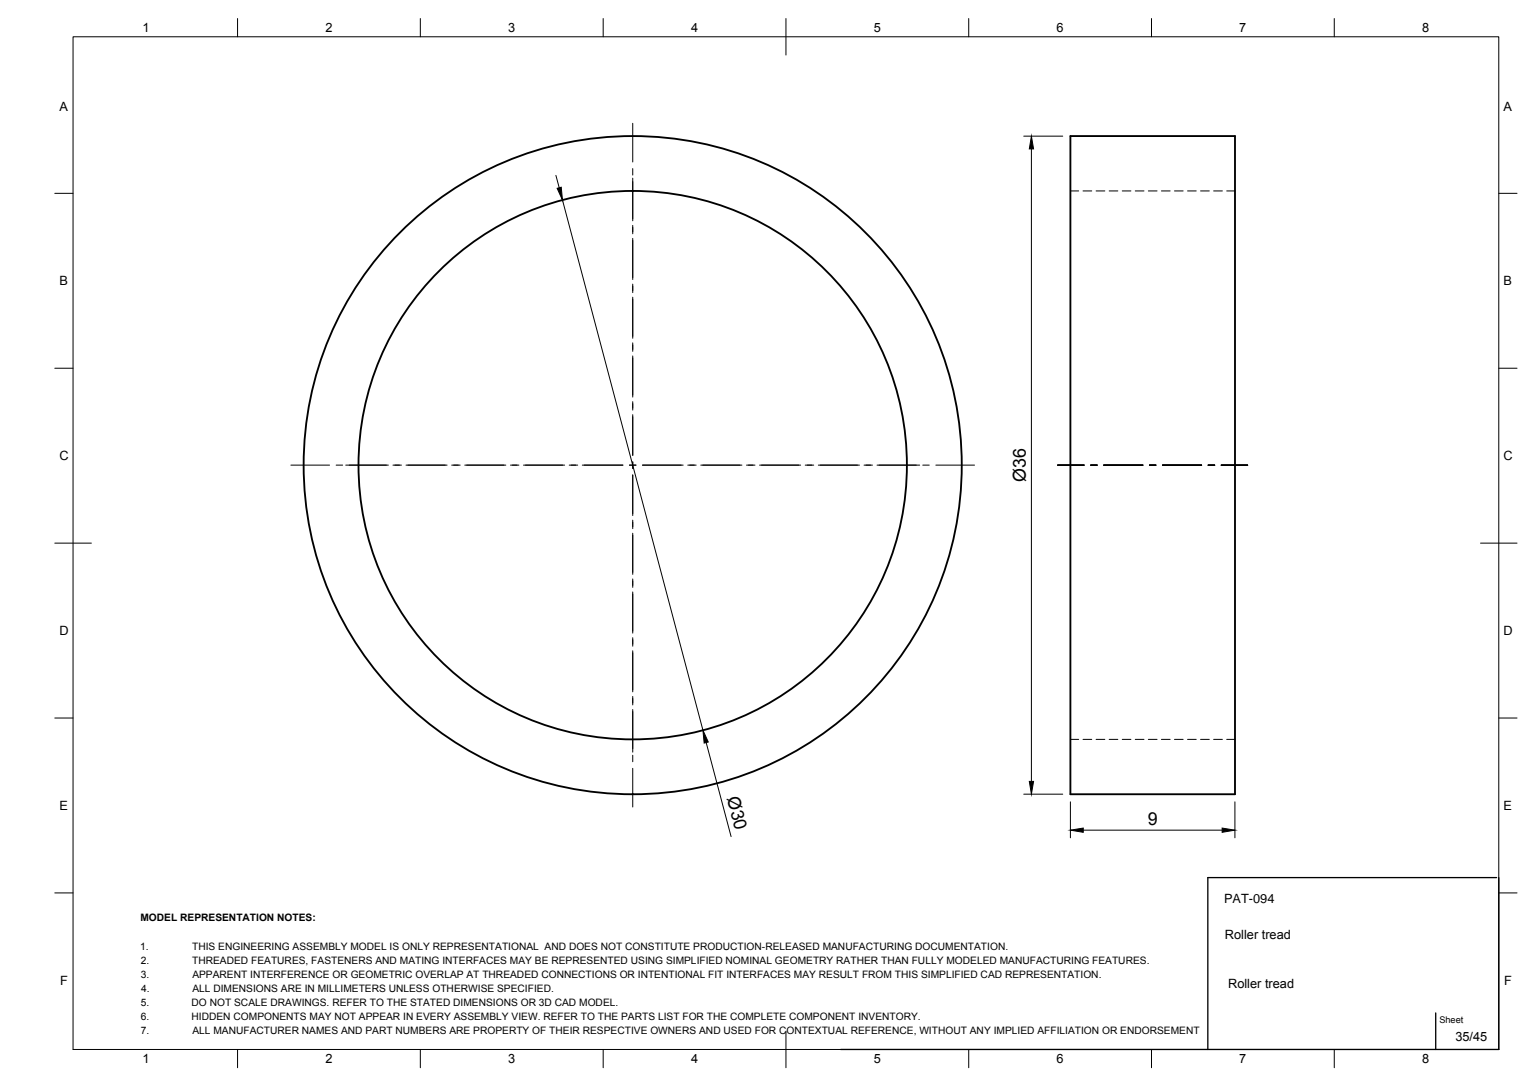
ISO-10303-21;
HEADER;
/* Generated by software containing ST-Developer
 * from STEP Tools, Inc. (www.steptools.com) 
 */

FILE_DESCRIPTION(
/* description */ ('Shaft runout checking stand'),
/* implementation_level */ '2;1');

FILE_NAME(
/* name */ 'Roller tread.step',
/* time_stamp */ '2026-11-02T21:12:33-08:00',
/* author */ (''),
/* organization */ (''),
/* preprocessor_version */ 'ST-DEVELOPER v20.2',
/* originating_system */ 'Autodesk Translation Framework v15.17.0.0',
/* authorisation */ '');

FILE_SCHEMA (('AUTOMOTIVE_DESIGN { 1 0 10303 214 3 1 1 }'));
ENDSEC;

DATA;
#10=MECHANICAL_DESIGN_GEOMETRIC_PRESENTATION_REPRESENTATION('',(#511),#11748);
#417=SHAPE_REPRESENTATION_RELATIONSHIP('SRR','None',#11969,#460);
#460=ADVANCED_BREP_SHAPE_REPRESENTATION('',(#559),#11745);
#511=STYLED_ITEM('',(#12169),#559);
#559=MANIFOLD_SOLID_BREP('Body1',#6257);
#667=FACE_BOUND('',#1870,.T.);
#668=FACE_BOUND('',#1872,.T.);
#926=CIRCLE('',#7457,1.5);
#927=CIRCLE('',#7458,1.5);
#928=CIRCLE('',#7460,1.8);
#929=CIRCLE('',#7461,1.8);
#1032=CYLINDRICAL_SURFACE('',#7456,1.5);
#1033=CYLINDRICAL_SURFACE('',#7459,1.8);
#1394=FACE_OUTER_BOUND('',#1867,.T.);
#1395=FACE_OUTER_BOUND('',#1868,.T.);
#1396=FACE_OUTER_BOUND('',#1869,.T.);
#1397=FACE_OUTER_BOUND('',#1871,.T.);
#1867=EDGE_LOOP('',(#5568,#5569,#5570,#5571));
#1868=EDGE_LOOP('',(#5572,#5573,#5574,#5575));
#1869=EDGE_LOOP('',(#5576));
#1870=EDGE_LOOP('',(#5577));
#1871=EDGE_LOOP('',(#5578));
#1872=EDGE_LOOP('',(#5579));
#2346=LINE('',#11601,#2813);
#2347=LINE('',#11607,#2814);
#2813=VECTOR('',#9401,1.5);
#2814=VECTOR('',#9408,1.8);
#3318=VERTEX_POINT('',#11598);
#3319=VERTEX_POINT('',#11600);
#3320=VERTEX_POINT('',#11604);
#3321=VERTEX_POINT('',#11606);
#4070=EDGE_CURVE('',#3318,#3318,#926,.T.);
#4071=EDGE_CURVE('',#3318,#3319,#2346,.T.);
#4072=EDGE_CURVE('',#3319,#3319,#927,.T.);
#4073=EDGE_CURVE('',#3320,#3320,#928,.T.);
#4074=EDGE_CURVE('',#3320,#3321,#2347,.T.);
#4075=EDGE_CURVE('',#3321,#3321,#929,.T.);
#5568=ORIENTED_EDGE('',*,*,#4070,.F.);
#5569=ORIENTED_EDGE('',*,*,#4071,.T.);
#5570=ORIENTED_EDGE('',*,*,#4072,.T.);
#5571=ORIENTED_EDGE('',*,*,#4071,.F.);
#5572=ORIENTED_EDGE('',*,*,#4073,.F.);
#5573=ORIENTED_EDGE('',*,*,#4074,.T.);
#5574=ORIENTED_EDGE('',*,*,#4075,.T.);
#5575=ORIENTED_EDGE('',*,*,#4074,.F.);
#5576=ORIENTED_EDGE('',*,*,#4073,.T.);
#5577=ORIENTED_EDGE('',*,*,#4070,.T.);
#5578=ORIENTED_EDGE('',*,*,#4075,.F.);
#5579=ORIENTED_EDGE('',*,*,#4072,.F.);
#5832=PLANE('',#7462);
#5833=PLANE('',#7463);
#6194=ADVANCED_FACE('',(#1394),#1032,.F.);
#6195=ADVANCED_FACE('',(#1395),#1033,.T.);
#6196=ADVANCED_FACE('',(#1396,#667),#5832,.T.);
#6197=ADVANCED_FACE('',(#1397,#668),#5833,.F.);
#6257=CLOSED_SHELL('',(#6194,#6195,#6196,#6197));
#7455=AXIS2_PLACEMENT_3D('',#11596,#9395,#9396);
#7456=AXIS2_PLACEMENT_3D('',#11597,#9397,#9398);
#7457=AXIS2_PLACEMENT_3D('',#11599,#9399,#9400);
#7458=AXIS2_PLACEMENT_3D('',#11602,#9402,#9403);
#7459=AXIS2_PLACEMENT_3D('',#11603,#9404,#9405);
#7460=AXIS2_PLACEMENT_3D('',#11605,#9406,#9407);
#7461=AXIS2_PLACEMENT_3D('',#11608,#9409,#9410);
#7462=AXIS2_PLACEMENT_3D('',#11609,#9411,#9412);
#7463=AXIS2_PLACEMENT_3D('',#11610,#9413,#9414);
#9395=DIRECTION('axis',(0.,0.,1.));
#9396=DIRECTION('refdir',(1.,0.,0.));
#9397=DIRECTION('center_axis',(0.,1.,0.));
#9398=DIRECTION('ref_axis',(1.,0.,0.));
#9399=DIRECTION('center_axis',(0.,-1.,0.));
#9400=DIRECTION('ref_axis',(1.,0.,0.));
#9401=DIRECTION('',(0.,-1.,0.));
#9402=DIRECTION('center_axis',(0.,-1.,0.));
#9403=DIRECTION('ref_axis',(1.,0.,0.));
#9404=DIRECTION('center_axis',(0.,1.,0.));
#9405=DIRECTION('ref_axis',(1.,0.,0.));
#9406=DIRECTION('center_axis',(0.,1.,0.));
#9407=DIRECTION('ref_axis',(1.,0.,0.));
#9408=DIRECTION('',(0.,-1.,0.));
#9409=DIRECTION('center_axis',(0.,1.,0.));
#9410=DIRECTION('ref_axis',(1.,0.,0.));
#9411=DIRECTION('center_axis',(0.,1.,0.));
#9412=DIRECTION('ref_axis',(1.,0.,0.));
#9413=DIRECTION('center_axis',(0.,1.,0.));
#9414=DIRECTION('ref_axis',(1.,0.,0.));
#11596=CARTESIAN_POINT('',(0.,0.,0.));
#11597=CARTESIAN_POINT('Origin',(-2.,-10.45,5.));
#11598=CARTESIAN_POINT('',(-3.5,-9.55,5.));
#11599=CARTESIAN_POINT('Origin',(-2.,-9.55,5.));
#11600=CARTESIAN_POINT('',(-3.5,-10.45,5.));
#11601=CARTESIAN_POINT('',(-3.5,-10.45,5.));
#11602=CARTESIAN_POINT('Origin',(-2.,-10.45,5.));
#11603=CARTESIAN_POINT('Origin',(-2.,-10.45,5.));
#11604=CARTESIAN_POINT('',(-3.8,-9.55,5.));
#11605=CARTESIAN_POINT('Origin',(-2.,-9.55,5.));
#11606=CARTESIAN_POINT('',(-3.8,-10.45,5.));
#11607=CARTESIAN_POINT('',(-3.8,-10.45,5.));
#11608=CARTESIAN_POINT('Origin',(-2.,-10.45,5.));
#11609=CARTESIAN_POINT('Origin',(-2.,-9.55,5.));
#11610=CARTESIAN_POINT('Origin',(-2.,-10.45,5.));
#11696=UNCERTAINTY_MEASURE_WITH_UNIT(LENGTH_MEASURE(0.001),#11749,
'DISTANCE_ACCURACY_VALUE',
'Maximum model space distance between geometric entities at asserted c
onnectivities');
#11699=UNCERTAINTY_MEASURE_WITH_UNIT(LENGTH_MEASURE(0.001),#11749,
'DISTANCE_ACCURACY_VALUE',
'Maximum model space distance between geometric entities at asserted c
onnectivities');
#11745=(
GEOMETRIC_REPRESENTATION_CONTEXT(3)
GLOBAL_UNCERTAINTY_ASSIGNED_CONTEXT((#11696))
GLOBAL_UNIT_ASSIGNED_CONTEXT((#11749,#11751,#11752))
REPRESENTATION_CONTEXT('','3D')
);
#11748=(
GEOMETRIC_REPRESENTATION_CONTEXT(3)
GLOBAL_UNCERTAINTY_ASSIGNED_CONTEXT((#11699))
GLOBAL_UNIT_ASSIGNED_CONTEXT((#11749,#11751,#11752))
REPRESENTATION_CONTEXT('','3D')
);
#11749=(
LENGTH_UNIT()
NAMED_UNIT(*)
SI_UNIT(.CENTI.,.METRE.)
);
#11751=(
NAMED_UNIT(*)
PLANE_ANGLE_UNIT()
SI_UNIT($,.RADIAN.)
);
#11752=(
NAMED_UNIT(*)
SI_UNIT($,.STERADIAN.)
SOLID_ANGLE_UNIT()
);
#11798=SHAPE_DEFINITION_REPRESENTATION(#11911,#11969);
#11911=PRODUCT_DEFINITION_SHAPE('',$,#12018);
#11969=SHAPE_REPRESENTATION('',(#7455),#11745);
#11972=PRODUCT_DEFINITION_CONTEXT('part definition',#12118,'design');
#12018=PRODUCT_DEFINITION('Roller tread','Roller tread',#12066,#11972);
#12066=PRODUCT_DEFINITION_FORMATION('',$,#12165);
#12118=APPLICATION_CONTEXT(
'Core Data for Automotive Mechanical Design Process');
#12119=PRODUCT_CONTEXT('part definition',#12118,'mechanical');
#12165=PRODUCT('Roller tread','Roller tread','Roller tread',(#12119));
#12169=PRESENTATION_STYLE_ASSIGNMENT((#12174));
#12174=SURFACE_STYLE_USAGE(.BOTH.,#12179);
#12179=SURFACE_SIDE_STYLE('',(#12184));
#12184=SURFACE_STYLE_FILL_AREA(#12189);
#12189=FILL_AREA_STYLE('CAD Library Painted - Engineering blue',(#12194));
#12194=FILL_AREA_STYLE_COLOUR('CAD Library Painted - Engineering blue',
#12199);
#12199=COLOUR_RGB('CAD Library Painted - Engineering blue',0.12156862745098,
0.356862745098039,0.6);
ENDSEC;
END-ISO-10303-21;
